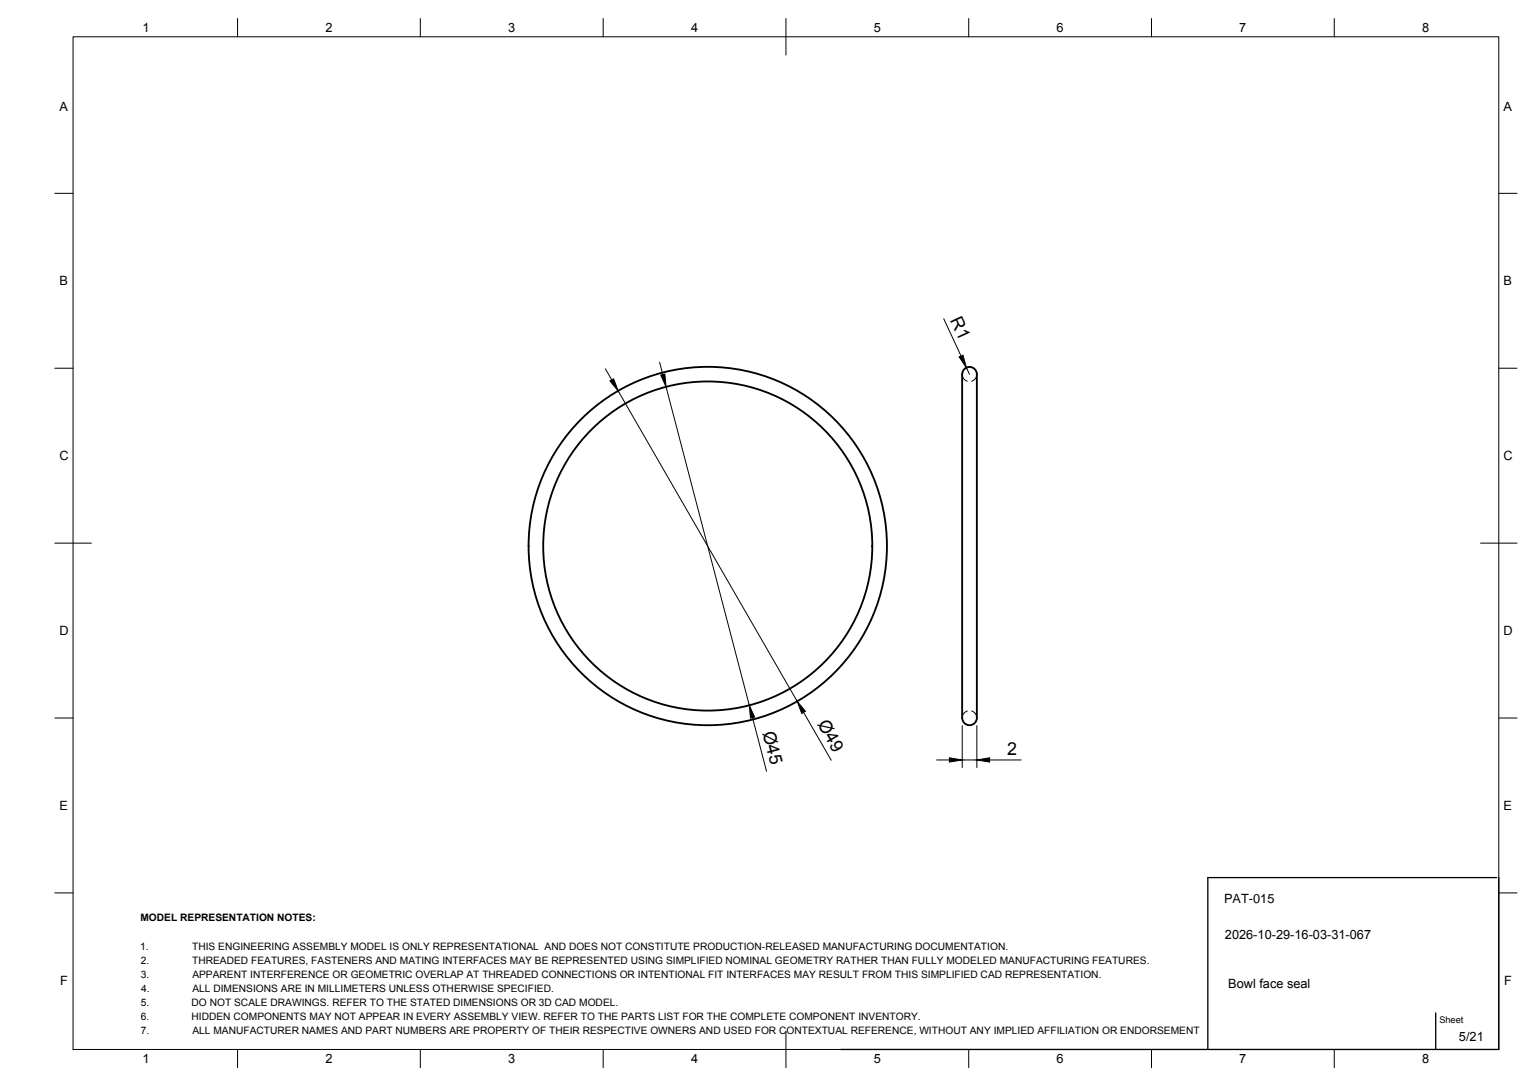
ISO-10303-21;
HEADER;
/* Generated by software containing ST-Developer
 * from STEP Tools, Inc. (www.steptools.com) 
 */

FILE_DESCRIPTION(
/* description */ ('PAT-015'),
/* implementation_level */ '2;1');

FILE_NAME(
/* name */ 'Bowl face seal.step',
/* time_stamp */ '2026-10-29T16:03:43-07:00',
/* author */ (''),
/* organization */ (''),
/* preprocessor_version */ 'ST-DEVELOPER v20.2',
/* originating_system */ 'Autodesk Translation Framework v15.17.0.0',
/* authorisation */ '');

FILE_SCHEMA (('AUTOMOTIVE_DESIGN { 1 0 10303 214 3 1 1 }'));
ENDSEC;

DATA;
#10=MECHANICAL_DESIGN_GEOMETRIC_PRESENTATION_REPRESENTATION('',(#231),#10266);
#182=TOROIDAL_SURFACE('',#5115,2.35,0.1);
#185=SHAPE_REPRESENTATION_RELATIONSHIP('SRR','None',#10356,#208);
#208=ADVANCED_BREP_SHAPE_REPRESENTATION('',(#256),#10244);
#231=STYLED_ITEM('',(#10554),#256);
#256=MANIFOLD_SOLID_BREP('Body1',#4690);
#637=FACE_OUTER_BOUND('',#953,.T.);
#953=EDGE_LOOP('',(#3363,#3364,#3365,#3366));
#1945=CIRCLE('',#5116,0.1);
#1946=CIRCLE('',#5117,2.25);
#2200=VERTEX_POINT('',#7511);
#2637=EDGE_CURVE('',#2200,#2200,#1945,.T.);
#2638=EDGE_CURVE('',#2200,#2200,#1946,.T.);
#3363=ORIENTED_EDGE('',*,*,#2637,.F.);
#3364=ORIENTED_EDGE('',*,*,#2638,.T.);
#3365=ORIENTED_EDGE('',*,*,#2637,.T.);
#3366=ORIENTED_EDGE('',*,*,#2638,.F.);
#4472=ADVANCED_FACE('',(#637),#182,.T.);
#4690=CLOSED_SHELL('',(#4472));
#5114=AXIS2_PLACEMENT_3D('',#7509,#5887,#5888);
#5115=AXIS2_PLACEMENT_3D('',#7510,#5889,#5890);
#5116=AXIS2_PLACEMENT_3D('',#7512,#5891,#5892);
#5117=AXIS2_PLACEMENT_3D('',#7513,#5893,#5894);
#5887=DIRECTION('axis',(0.,0.,1.));
#5888=DIRECTION('refdir',(1.,0.,0.));
#5889=DIRECTION('center_axis',(0.,0.,1.));
#5890=DIRECTION('ref_axis',(1.,0.,0.));
#5891=DIRECTION('center_axis',(1.22464679914735E-16,-1.,0.));
#5892=DIRECTION('ref_axis',(-1.,-1.22464679914735E-16,0.));
#5893=DIRECTION('center_axis',(0.,0.,-1.));
#5894=DIRECTION('ref_axis',(1.,0.,0.));
#7509=CARTESIAN_POINT('',(0.,0.,0.));
#7510=CARTESIAN_POINT('Origin',(0.,0.,1.4));
#7511=CARTESIAN_POINT('',(-2.25,-2.75545529808154E-16,1.4));
#7512=CARTESIAN_POINT('Origin',(-2.35,-2.87791997799628E-16,1.4));
#7513=CARTESIAN_POINT('Origin',(0.,0.,1.4));
#10219=UNCERTAINTY_MEASURE_WITH_UNIT(LENGTH_MEASURE(0.001),#10267,
'DISTANCE_ACCURACY_VALUE',
'Maximum model space distance between geometric entities at asserted c
onnectivities');
#10241=UNCERTAINTY_MEASURE_WITH_UNIT(LENGTH_MEASURE(0.001),#10267,
'DISTANCE_ACCURACY_VALUE',
'Maximum model space distance between geometric entities at asserted c
onnectivities');
#10244=(
GEOMETRIC_REPRESENTATION_CONTEXT(3)
GLOBAL_UNCERTAINTY_ASSIGNED_CONTEXT((#10219))
GLOBAL_UNIT_ASSIGNED_CONTEXT((#10267,#10269,#10270))
REPRESENTATION_CONTEXT('','3D')
);
#10266=(
GEOMETRIC_REPRESENTATION_CONTEXT(3)
GLOBAL_UNCERTAINTY_ASSIGNED_CONTEXT((#10241))
GLOBAL_UNIT_ASSIGNED_CONTEXT((#10267,#10269,#10270))
REPRESENTATION_CONTEXT('','3D')
);
#10267=(
LENGTH_UNIT()
NAMED_UNIT(*)
SI_UNIT(.CENTI.,.METRE.)
);
#10269=(
NAMED_UNIT(*)
PLANE_ANGLE_UNIT()
SI_UNIT($,.RADIAN.)
);
#10270=(
NAMED_UNIT(*)
SI_UNIT($,.STERADIAN.)
SOLID_ANGLE_UNIT()
);
#10273=SHAPE_DEFINITION_REPRESENTATION(#10297,#10356);
#10297=PRODUCT_DEFINITION_SHAPE('',$,#10381);
#10356=SHAPE_REPRESENTATION('',(#5114),#10244);
#10378=PRODUCT_DEFINITION_CONTEXT('part definition',#10452,'design');
#10381=PRODUCT_DEFINITION('Bowl face seal','Bowl face seal',#10405,
#10378);
#10405=PRODUCT_DEFINITION_FORMATION('',$,#10456);
#10452=APPLICATION_CONTEXT(
'Core Data for Automotive Mechanical Design Process');
#10453=PRODUCT_CONTEXT('part definition',#10452,'mechanical');
#10456=PRODUCT('Bowl face seal','Bowl face seal',
'Bowl face seal',(#10453));
#10548=COLOUR_RGB('Black',0.12,0.14,0.17);
#10549=FILL_AREA_STYLE_COLOUR('',#10548);
#10550=FILL_AREA_STYLE('',(#10549));
#10551=SURFACE_STYLE_FILL_AREA(#10550);
#10552=SURFACE_SIDE_STYLE('',(#10551));
#10553=SURFACE_STYLE_USAGE(.BOTH.,#10552);
#10554=PRESENTATION_STYLE_ASSIGNMENT((#10553));
ENDSEC;
END-ISO-10303-21;
